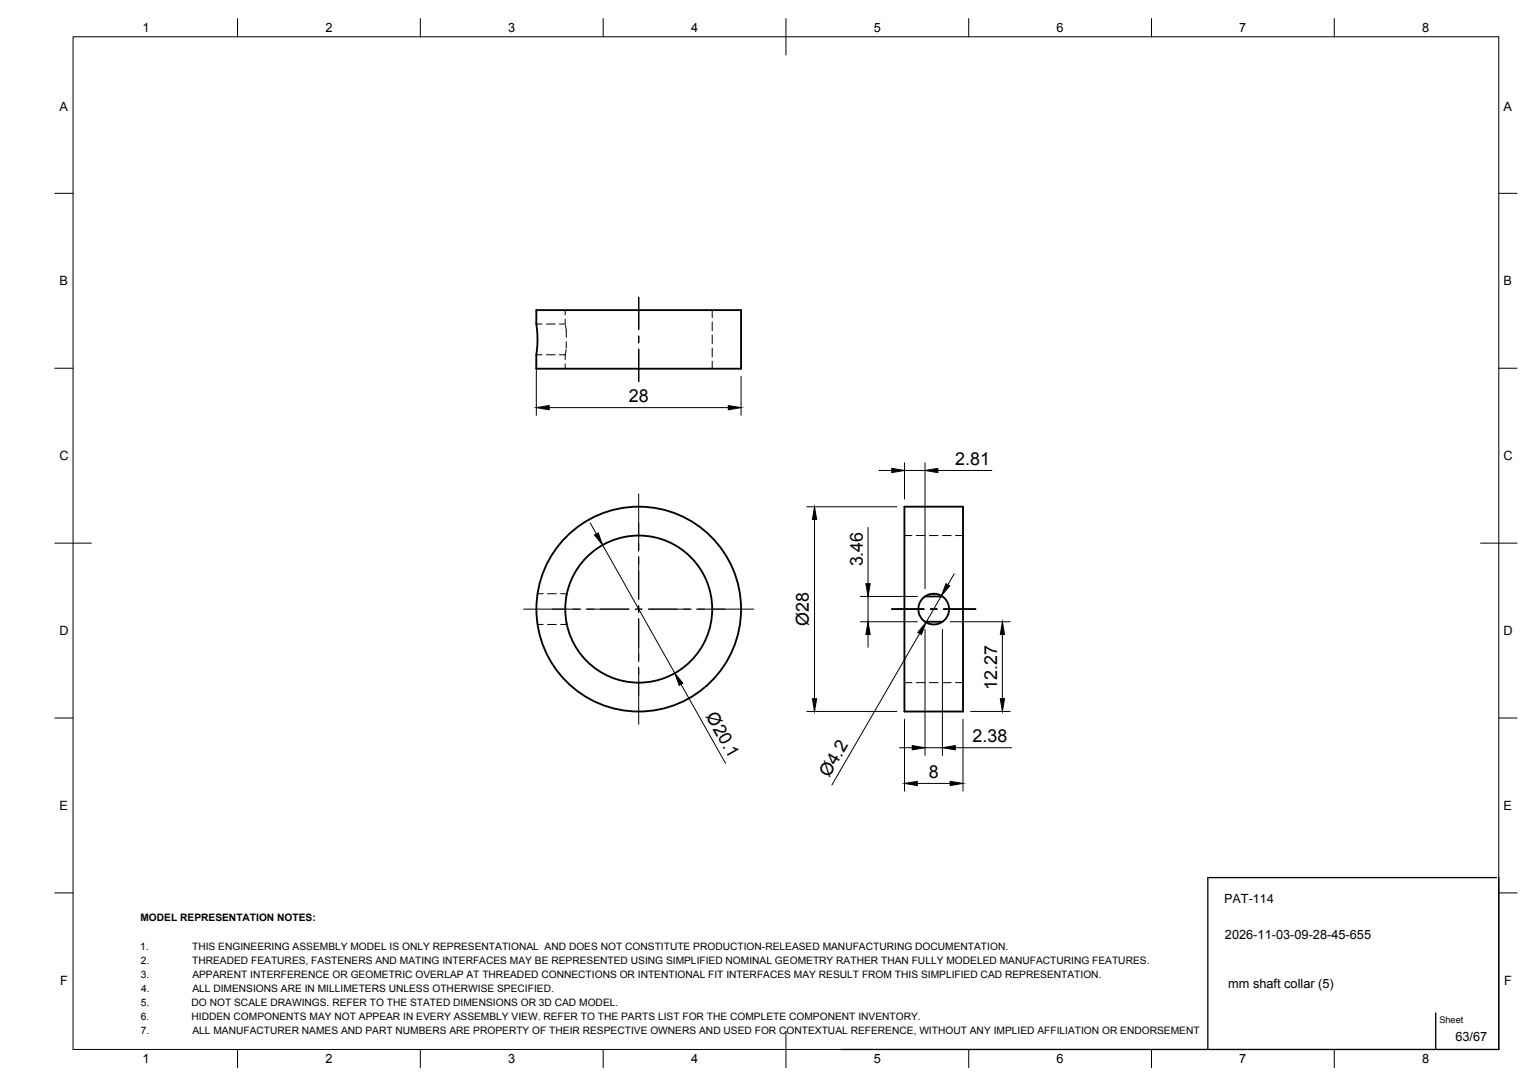
ISO-10303-21;
HEADER;
/* Generated by software containing ST-Developer
 * from STEP Tools, Inc. (www.steptools.com) 
 */

FILE_DESCRIPTION(
/* description */ ('Two-stage gear reducer in split housing'),
/* implementation_level */ '2;1');

FILE_NAME(
/* name */ 'mm shaft collar (5).step',
/* time_stamp */ '2026-10-28T03:22:31-07:00',
/* author */ (''),
/* organization */ (''),
/* preprocessor_version */ 'ST-DEVELOPER v20.2',
/* originating_system */ 'Autodesk Translation Framework v15.17.0.0',
/* authorisation */ '');

FILE_SCHEMA (('AUTOMOTIVE_DESIGN { 1 0 10303 214 3 1 1 }'));
ENDSEC;

DATA;
#10=MECHANICAL_DESIGN_GEOMETRIC_PRESENTATION_REPRESENTATION('',(#1297),#73366);
#983=B_SPLINE_CURVE_WITH_KNOTS('',3,(#49393,#49394,#49395,#49396,#49397,
#49398,#49399,#49400,#49401,#49402,#49403,#49404,#49405,#49406),
 .UNSPECIFIED.,.F.,.F.,(4,2,2,2,2,2,4),(0.756005737987027,0.79356882756465,
0.872922520054205,0.95227621254376,1.03162990503331,1.11098359752287,1.14854668710049),
 .UNSPECIFIED.);
#984=B_SPLINE_CURVE_WITH_KNOTS('',3,(#49412,#49413,#49414,#49415,#49416,
#49417,#49418,#49419,#49420,#49421,#49422,#49423,#49424,#49425,#49426,#49427,
#49428,#49429),.UNSPECIFIED.,.F.,.F.,(4,2,2,2,2,2,2,2,4),(0.,0.0792334805614376,
0.158466961122875,0.237699060165218,0.316931159207561,0.396163258249904,
0.475395357292247,0.554628837853685,0.633862318415122),.UNSPECIFIED.);
#985=B_SPLINE_CURVE_WITH_KNOTS('',3,(#49430,#49431,#49432,#49433,#49434,
#49435,#49436,#49437,#49438,#49439,#49440,#49441,#49442,#49443,#49444,#49445,
#49446,#49447),.UNSPECIFIED.,.F.,.F.,(4,2,2,2,2,2,2,2,4),(0.633862318415122,
0.71309579897656,0.792329279537998,0.871561378580341,0.950793477622684,
1.03002557666503,1.10925767570737,1.18849115626881,1.26772463683024),
 .UNSPECIFIED.);
#986=B_SPLINE_CURVE_WITH_KNOTS('',3,(#49450,#49451,#49452,#49453,#49454,
#49455,#49456,#49457,#49458,#49459,#49460,#49461,#49462,#49463),
 .UNSPECIFIED.,.F.,.F.,(4,2,2,2,2,2,4),(0.121154929624521,0.158718019202143,
0.238071711691698,0.317425404181253,0.396779096670808,0.476132789160363,
0.513695878737991),.UNSPECIFIED.);
#1170=SHAPE_REPRESENTATION_RELATIONSHIP('SRR','None',#73662,#1226);
#1226=ADVANCED_BREP_SHAPE_REPRESENTATION('',(#1366),#73358);
#1297=STYLED_ITEM('',(#73988),#1366);
#1366=MANIFOLD_SOLID_BREP('Body1',#16187);
#1586=FACE_BOUND('',#3831,.T.);
#1587=FACE_BOUND('',#3833,.T.);
#1588=FACE_BOUND('',#3835,.T.);
#1589=FACE_BOUND('',#3837,.T.);
#1925=PLANE('',#18167);
#1926=PLANE('',#18172);
#1927=PLANE('',#18179);
#1928=PLANE('',#18180);
#2702=FACE_OUTER_BOUND('',#3827,.T.);
#2703=FACE_OUTER_BOUND('',#3828,.T.);
#2704=FACE_OUTER_BOUND('',#3829,.T.);
#2705=FACE_OUTER_BOUND('',#3830,.T.);
#2706=FACE_OUTER_BOUND('',#3832,.T.);
#2707=FACE_OUTER_BOUND('',#3834,.T.);
#2708=FACE_OUTER_BOUND('',#3836,.T.);
#3827=EDGE_LOOP('',(#13739,#13740));
#3828=EDGE_LOOP('',(#13741,#13742,#13743,#13744,#13745,#13746,#13747,#13748,
#13749));
#3829=EDGE_LOOP('',(#13750,#13751,#13752));
#3830=EDGE_LOOP('',(#13753,#13754,#13755,#13756));
#3831=EDGE_LOOP('',(#13757,#13758,#13759,#13760));
#3832=EDGE_LOOP('',(#13761,#13762,#13763,#13764));
#3833=EDGE_LOOP('',(#13765,#13766));
#3834=EDGE_LOOP('',(#13767));
#3835=EDGE_LOOP('',(#13768));
#3836=EDGE_LOOP('',(#13769));
#3837=EDGE_LOOP('',(#13770));
#4851=LINE('',#49389,#5875);
#4852=LINE('',#49410,#5876);
#4853=LINE('',#49465,#5877);
#4854=LINE('',#49470,#5878);
#4855=LINE('',#49476,#5879);
#5875=VECTOR('',#21965,1.);
#5876=VECTOR('',#21972,0.210000000000001);
#5877=VECTOR('',#21977,1.);
#5878=VECTOR('',#21982,1.005);
#5879=VECTOR('',#21989,1.4);
#6713=CIRCLE('',#18168,0.210000000000001);
#6714=CIRCLE('',#18170,0.210000000000001);
#6715=CIRCLE('',#18171,0.210000000000001);
#6716=CIRCLE('',#18174,1.005);
#6717=CIRCLE('',#18175,1.005);
#6718=CIRCLE('',#18177,1.4);
#6719=CIRCLE('',#18178,1.4);
#7918=VERTEX_POINT('',#49387);
#7919=VERTEX_POINT('',#49388);
#7920=VERTEX_POINT('',#49392);
#7921=VERTEX_POINT('',#49407);
#7922=VERTEX_POINT('',#49409);
#7923=VERTEX_POINT('',#49411);
#7924=VERTEX_POINT('',#49448);
#7925=VERTEX_POINT('',#49467);
#7926=VERTEX_POINT('',#49469);
#7927=VERTEX_POINT('',#49473);
#7928=VERTEX_POINT('',#49475);
#9923=EDGE_CURVE('',#7918,#7919,#4851,.T.);
#9924=EDGE_CURVE('',#7918,#7919,#6713,.T.);
#9925=EDGE_CURVE('',#7920,#7918,#983,.T.);
#9926=EDGE_CURVE('',#7921,#7920,#6714,.T.);
#9927=EDGE_CURVE('',#7921,#7922,#4852,.T.);
#9928=EDGE_CURVE('',#7923,#7922,#984,.T.);
#9929=EDGE_CURVE('',#7922,#7923,#985,.T.);
#9930=EDGE_CURVE('',#7924,#7921,#6715,.T.);
#9931=EDGE_CURVE('',#7919,#7924,#986,.T.);
#9932=EDGE_CURVE('',#7924,#7920,#4853,.T.);
#9933=EDGE_CURVE('',#7925,#7925,#6716,.T.);
#9934=EDGE_CURVE('',#7925,#7926,#4854,.T.);
#9935=EDGE_CURVE('',#7926,#7926,#6717,.T.);
#9936=EDGE_CURVE('',#7927,#7927,#6718,.T.);
#9937=EDGE_CURVE('',#7927,#7928,#4855,.T.);
#9938=EDGE_CURVE('',#7928,#7928,#6719,.T.);
#13739=ORIENTED_EDGE('',*,*,#9923,.F.);
#13740=ORIENTED_EDGE('',*,*,#9924,.T.);
#13741=ORIENTED_EDGE('',*,*,#9925,.F.);
#13742=ORIENTED_EDGE('',*,*,#9926,.F.);
#13743=ORIENTED_EDGE('',*,*,#9927,.T.);
#13744=ORIENTED_EDGE('',*,*,#9928,.F.);
#13745=ORIENTED_EDGE('',*,*,#9929,.F.);
#13746=ORIENTED_EDGE('',*,*,#9927,.F.);
#13747=ORIENTED_EDGE('',*,*,#9930,.F.);
#13748=ORIENTED_EDGE('',*,*,#9931,.F.);
#13749=ORIENTED_EDGE('',*,*,#9924,.F.);
#13750=ORIENTED_EDGE('',*,*,#9932,.F.);
#13751=ORIENTED_EDGE('',*,*,#9930,.T.);
#13752=ORIENTED_EDGE('',*,*,#9926,.T.);
#13753=ORIENTED_EDGE('',*,*,#9933,.F.);
#13754=ORIENTED_EDGE('',*,*,#9934,.T.);
#13755=ORIENTED_EDGE('',*,*,#9935,.T.);
#13756=ORIENTED_EDGE('',*,*,#9934,.F.);
#13757=ORIENTED_EDGE('',*,*,#9931,.T.);
#13758=ORIENTED_EDGE('',*,*,#9932,.T.);
#13759=ORIENTED_EDGE('',*,*,#9925,.T.);
#13760=ORIENTED_EDGE('',*,*,#9923,.T.);
#13761=ORIENTED_EDGE('',*,*,#9936,.F.);
#13762=ORIENTED_EDGE('',*,*,#9937,.T.);
#13763=ORIENTED_EDGE('',*,*,#9938,.T.);
#13764=ORIENTED_EDGE('',*,*,#9937,.F.);
#13765=ORIENTED_EDGE('',*,*,#9928,.T.);
#13766=ORIENTED_EDGE('',*,*,#9929,.T.);
#13767=ORIENTED_EDGE('',*,*,#9936,.T.);
#13768=ORIENTED_EDGE('',*,*,#9933,.T.);
#13769=ORIENTED_EDGE('',*,*,#9938,.F.);
#13770=ORIENTED_EDGE('',*,*,#9935,.F.);
#15155=CYLINDRICAL_SURFACE('',#18169,0.210000000000001);
#15156=CYLINDRICAL_SURFACE('',#18173,1.005);
#15157=CYLINDRICAL_SURFACE('',#18176,1.4);
#15909=ADVANCED_FACE('',(#2702),#1925,.T.);
#15910=ADVANCED_FACE('',(#2703),#15155,.F.);
#15911=ADVANCED_FACE('',(#2704),#1926,.T.);
#15912=ADVANCED_FACE('',(#2705,#1586),#15156,.F.);
#15913=ADVANCED_FACE('',(#2706,#1587),#15157,.T.);
#15914=ADVANCED_FACE('',(#2707,#1588),#1927,.T.);
#15915=ADVANCED_FACE('',(#2708,#1589),#1928,.F.);
#16187=CLOSED_SHELL('',(#15909,#15910,#15911,#15912,#15913,#15914,#15915));
#18166=AXIS2_PLACEMENT_3D('',#49385,#21961,#21962);
#18167=AXIS2_PLACEMENT_3D('',#49386,#21963,#21964);
#18168=AXIS2_PLACEMENT_3D('',#49390,#21966,#21967);
#18169=AXIS2_PLACEMENT_3D('',#49391,#21968,#21969);
#18170=AXIS2_PLACEMENT_3D('',#49408,#21970,#21971);
#18171=AXIS2_PLACEMENT_3D('',#49449,#21973,#21974);
#18172=AXIS2_PLACEMENT_3D('',#49464,#21975,#21976);
#18173=AXIS2_PLACEMENT_3D('',#49466,#21978,#21979);
#18174=AXIS2_PLACEMENT_3D('',#49468,#21980,#21981);
#18175=AXIS2_PLACEMENT_3D('',#49471,#21983,#21984);
#18176=AXIS2_PLACEMENT_3D('',#49472,#21985,#21986);
#18177=AXIS2_PLACEMENT_3D('',#49474,#21987,#21988);
#18178=AXIS2_PLACEMENT_3D('',#49477,#21990,#21991);
#18179=AXIS2_PLACEMENT_3D('',#49478,#21992,#21993);
#18180=AXIS2_PLACEMENT_3D('',#49479,#21994,#21995);
#21961=DIRECTION('axis',(0.,0.,1.));
#21962=DIRECTION('refdir',(1.,0.,0.));
#21963=DIRECTION('center_axis',(0.,0.,1.));
#21964=DIRECTION('ref_axis',(1.,0.,0.));
#21965=DIRECTION('',(0.,1.,0.));
#21966=DIRECTION('center_axis',(0.,0.,1.));
#21967=DIRECTION('ref_axis',(1.,0.,0.));
#21968=DIRECTION('center_axis',(0.,0.,1.));
#21969=DIRECTION('ref_axis',(1.,0.,0.));
#21970=DIRECTION('center_axis',(0.,0.,1.));
#21971=DIRECTION('ref_axis',(1.,0.,0.));
#21972=DIRECTION('',(0.,0.,1.));
#21973=DIRECTION('center_axis',(0.,0.,1.));
#21974=DIRECTION('ref_axis',(1.,0.,0.));
#21975=DIRECTION('center_axis',(0.,0.,1.));
#21976=DIRECTION('ref_axis',(1.,0.,0.));
#21977=DIRECTION('',(0.,-1.,0.));
#21978=DIRECTION('center_axis',(0.,1.,0.));
#21979=DIRECTION('ref_axis',(1.,0.,0.));
#21980=DIRECTION('center_axis',(0.,-1.,0.));
#21981=DIRECTION('ref_axis',(1.,0.,0.));
#21982=DIRECTION('',(0.,-1.,0.));
#21983=DIRECTION('center_axis',(0.,-1.,0.));
#21984=DIRECTION('ref_axis',(1.,0.,0.));
#21985=DIRECTION('center_axis',(0.,1.,0.));
#21986=DIRECTION('ref_axis',(1.,0.,0.));
#21987=DIRECTION('center_axis',(0.,1.,0.));
#21988=DIRECTION('ref_axis',(1.,0.,0.));
#21989=DIRECTION('',(0.,-1.,0.));
#21990=DIRECTION('center_axis',(0.,1.,0.));
#21991=DIRECTION('ref_axis',(1.,0.,0.));
#21992=DIRECTION('center_axis',(0.,1.,0.));
#21993=DIRECTION('ref_axis',(1.,0.,0.));
#21994=DIRECTION('center_axis',(0.,1.,0.));
#21995=DIRECTION('ref_axis',(1.,0.,0.));
#49385=CARTESIAN_POINT('',(0.,0.,0.));
#49386=CARTESIAN_POINT('Origin',(12.,8.2,10.99));
#49387=CARTESIAN_POINT('',(12.1729884389201,8.08094119100208,10.99));
#49388=CARTESIAN_POINT('',(12.1729884389201,8.31905880899792,10.99));
#49389=CARTESIAN_POINT('',(12.1729884389201,7.8,10.99));
#49390=CARTESIAN_POINT('Origin',(12.,8.2,10.99));
#49391=CARTESIAN_POINT('Origin',(12.,8.2,10.99));
#49392=CARTESIAN_POINT('',(11.8270115610799,8.08094119100208,10.99));
#49393=CARTESIAN_POINT('Ctrl Pts',(11.8270115610799,8.08094119100208,10.99));
#49394=CARTESIAN_POINT('Ctrl Pts',(11.8344051346887,8.0701985776047,10.9912919219764));
#49395=CARTESIAN_POINT('Ctrl Pts',(11.8427028612744,8.06031229062725,10.992653949439));
#49396=CARTESIAN_POINT('Ctrl Pts',(11.8701079261549,8.03290722574673,10.9967480843909));
#49397=CARTESIAN_POINT('Ctrl Pts',(11.8936698322407,8.01675794366705,10.9996958932764));
#49398=CARTESIAN_POINT('Ctrl Pts',(11.9453870953676,7.99530220603509,11.0038502947236));
#49399=CARTESIAN_POINT('Ctrl Pts',(11.9735487691701,7.99,11.005));
#49400=CARTESIAN_POINT('Ctrl Pts',(12.0264512308299,7.99,11.005));
#49401=CARTESIAN_POINT('Ctrl Pts',(12.0546129046324,7.99530220603509,11.0038502947236));
#49402=CARTESIAN_POINT('Ctrl Pts',(12.1063301677593,8.01675794366705,10.9996958932764));
#49403=CARTESIAN_POINT('Ctrl Pts',(12.1298920738451,8.03290722574673,10.9967480843909));
#49404=CARTESIAN_POINT('Ctrl Pts',(12.1572971387256,8.06031229062725,10.992653949439));
#49405=CARTESIAN_POINT('Ctrl Pts',(12.1655948653113,8.0701985776047,10.9912919219764));
#49406=CARTESIAN_POINT('Ctrl Pts',(12.1729884389201,8.08094119100208,10.99));
#49407=CARTESIAN_POINT('',(11.79,8.2,10.99));
#49408=CARTESIAN_POINT('Origin',(12.,8.2,10.99));
#49409=CARTESIAN_POINT('',(11.79,8.2,11.38416039533));
#49410=CARTESIAN_POINT('',(11.79,8.2,10.99));
#49411=CARTESIAN_POINT('',(12.21,8.2,11.38416039533));
#49412=CARTESIAN_POINT('Ctrl Pts',(12.21,8.2,11.38416039533));
#49413=CARTESIAN_POINT('Ctrl Pts',(12.21,8.17358883981285,11.38416039533));
#49414=CARTESIAN_POINT('Ctrl Pts',(12.2047135491119,8.1454449403829,11.3849944296993));
#49415=CARTESIAN_POINT('Ctrl Pts',(12.1832699958585,8.09371735000826,11.3879947099895));
#49416=CARTESIAN_POINT('Ctrl Pts',(12.1671150376064,8.07013018950807,11.3901162943626));
#49417=CARTESIAN_POINT('Ctrl Pts',(12.1298701351968,8.03288528709843,11.394089123191));
#49418=CARTESIAN_POINT('Ctrl Pts',(12.1062828345902,8.01673007414492,11.3962002442067));
#49419=CARTESIAN_POINT('Ctrl Pts',(12.0545547656039,7.99528633552708,11.3991765222353));
#49420=CARTESIAN_POINT('Ctrl Pts',(12.0264106996808,7.99,11.4));
#49421=CARTESIAN_POINT('Ctrl Pts',(11.9735893003192,7.99,11.4));
#49422=CARTESIAN_POINT('Ctrl Pts',(11.9454452343961,7.99528633552708,11.3991765222353));
#49423=CARTESIAN_POINT('Ctrl Pts',(11.8937171654098,8.01673007414492,11.3962002442067));
#49424=CARTESIAN_POINT('Ctrl Pts',(11.8701298648032,8.03288528709843,11.394089123191));
#49425=CARTESIAN_POINT('Ctrl Pts',(11.8328849623936,8.07013018950807,11.3901162943626));
#49426=CARTESIAN_POINT('Ctrl Pts',(11.8167300041415,8.09371735000826,11.3879947099895));
#49427=CARTESIAN_POINT('Ctrl Pts',(11.7952864508881,8.1454449403829,11.3849944296993));
#49428=CARTESIAN_POINT('Ctrl Pts',(11.79,8.17358883981285,11.38416039533));
#49429=CARTESIAN_POINT('Ctrl Pts',(11.79,8.2,11.38416039533));
#49430=CARTESIAN_POINT('Ctrl Pts',(11.79,8.2,11.38416039533));
#49431=CARTESIAN_POINT('Ctrl Pts',(11.79,8.22641116018714,11.38416039533));
#49432=CARTESIAN_POINT('Ctrl Pts',(11.7952864508881,8.2545550596171,11.3849944296993));
#49433=CARTESIAN_POINT('Ctrl Pts',(11.8167300041415,8.30628264999174,11.3879947099895));
#49434=CARTESIAN_POINT('Ctrl Pts',(11.8328849623936,8.32986981049192,11.3901162943626));
#49435=CARTESIAN_POINT('Ctrl Pts',(11.8701298648032,8.36711471290156,11.394089123191));
#49436=CARTESIAN_POINT('Ctrl Pts',(11.8937171654098,8.38326992585508,11.3962002442067));
#49437=CARTESIAN_POINT('Ctrl Pts',(11.9454452343961,8.40471366447292,11.3991765222353));
#49438=CARTESIAN_POINT('Ctrl Pts',(11.9735893003192,8.41,11.4));
#49439=CARTESIAN_POINT('Ctrl Pts',(12.0264106996808,8.41,11.4));
#49440=CARTESIAN_POINT('Ctrl Pts',(12.0545547656039,8.40471366447292,11.3991765222353));
#49441=CARTESIAN_POINT('Ctrl Pts',(12.1062828345902,8.38326992585508,11.3962002442067));
#49442=CARTESIAN_POINT('Ctrl Pts',(12.1298701351968,8.36711471290156,11.394089123191));
#49443=CARTESIAN_POINT('Ctrl Pts',(12.1671150376064,8.32986981049192,11.3901162943626));
#49444=CARTESIAN_POINT('Ctrl Pts',(12.1832699958585,8.30628264999174,11.3879947099895));
#49445=CARTESIAN_POINT('Ctrl Pts',(12.2047135491119,8.2545550596171,11.3849944296993));
#49446=CARTESIAN_POINT('Ctrl Pts',(12.21,8.22641116018714,11.38416039533));
#49447=CARTESIAN_POINT('Ctrl Pts',(12.21,8.2,11.38416039533));
#49448=CARTESIAN_POINT('',(11.8270115610799,8.31905880899792,10.99));
#49449=CARTESIAN_POINT('Origin',(12.,8.2,10.99));
#49450=CARTESIAN_POINT('Ctrl Pts',(12.1729884389201,8.31905880899792,10.99));
#49451=CARTESIAN_POINT('Ctrl Pts',(12.1655948653113,8.32980142239529,10.9912919219764));
#49452=CARTESIAN_POINT('Ctrl Pts',(12.1572971387256,8.33968770937275,10.992653949439));
#49453=CARTESIAN_POINT('Ctrl Pts',(12.1298920738451,8.36709277425327,10.9967480843909));
#49454=CARTESIAN_POINT('Ctrl Pts',(12.1063301677593,8.38324205633295,10.9996958932764));
#49455=CARTESIAN_POINT('Ctrl Pts',(12.0546129046324,8.40469779396491,11.0038502947236));
#49456=CARTESIAN_POINT('Ctrl Pts',(12.0264512308299,8.41,11.005));
#49457=CARTESIAN_POINT('Ctrl Pts',(11.9735487691701,8.41,11.005));
#49458=CARTESIAN_POINT('Ctrl Pts',(11.9453870953676,8.40469779396491,11.0038502947236));
#49459=CARTESIAN_POINT('Ctrl Pts',(11.8936698322407,8.38324205633295,10.9996958932764));
#49460=CARTESIAN_POINT('Ctrl Pts',(11.8701079261549,8.36709277425327,10.9967480843909));
#49461=CARTESIAN_POINT('Ctrl Pts',(11.8427028612744,8.33968770937274,10.992653949439));
#49462=CARTESIAN_POINT('Ctrl Pts',(11.8344051346887,8.3298014223953,10.9912919219764));
#49463=CARTESIAN_POINT('Ctrl Pts',(11.8270115610799,8.31905880899792,10.99));
#49464=CARTESIAN_POINT('Origin',(12.,8.2,10.99));
#49465=CARTESIAN_POINT('',(11.8270115610799,7.8,10.99));
#49466=CARTESIAN_POINT('Origin',(12.,7.8,10.));
#49467=CARTESIAN_POINT('',(10.995,8.6,10.));
#49468=CARTESIAN_POINT('Origin',(12.,8.6,10.));
#49469=CARTESIAN_POINT('',(10.995,7.8,10.));
#49470=CARTESIAN_POINT('',(10.995,7.8,10.));
#49471=CARTESIAN_POINT('Origin',(12.,7.8,10.));
#49472=CARTESIAN_POINT('Origin',(12.,7.8,10.));
#49473=CARTESIAN_POINT('',(10.6,8.6,10.));
#49474=CARTESIAN_POINT('Origin',(12.,8.6,10.));
#49475=CARTESIAN_POINT('',(10.6,7.8,10.));
#49476=CARTESIAN_POINT('',(10.6,7.8,10.));
#49477=CARTESIAN_POINT('Origin',(12.,7.8,10.));
#49478=CARTESIAN_POINT('Origin',(12.,8.6,10.));
#49479=CARTESIAN_POINT('Origin',(12.,7.8,10.));
#73294=UNCERTAINTY_MEASURE_WITH_UNIT(LENGTH_MEASURE(0.001),#73367,
'DISTANCE_ACCURACY_VALUE',
'Maximum model space distance between geometric entities at asserted c
onnectivities');
#73302=UNCERTAINTY_MEASURE_WITH_UNIT(LENGTH_MEASURE(0.001),#73367,
'DISTANCE_ACCURACY_VALUE',
'Maximum model space distance between geometric entities at asserted c
onnectivities');
#73358=(
GEOMETRIC_REPRESENTATION_CONTEXT(3)
GLOBAL_UNCERTAINTY_ASSIGNED_CONTEXT((#73294))
GLOBAL_UNIT_ASSIGNED_CONTEXT((#73367,#73369,#73370))
REPRESENTATION_CONTEXT('','3D')
);
#73366=(
GEOMETRIC_REPRESENTATION_CONTEXT(3)
GLOBAL_UNCERTAINTY_ASSIGNED_CONTEXT((#73302))
GLOBAL_UNIT_ASSIGNED_CONTEXT((#73367,#73369,#73370))
REPRESENTATION_CONTEXT('','3D')
);
#73367=(
LENGTH_UNIT()
NAMED_UNIT(*)
SI_UNIT(.CENTI.,.METRE.)
);
#73369=(
NAMED_UNIT(*)
PLANE_ANGLE_UNIT()
SI_UNIT($,.RADIAN.)
);
#73370=(
NAMED_UNIT(*)
SI_UNIT($,.STERADIAN.)
SOLID_ANGLE_UNIT()
);
#73426=SHAPE_DEFINITION_REPRESENTATION(#73559,#73662);
#73559=PRODUCT_DEFINITION_SHAPE('',$,#73726);
#73662=SHAPE_REPRESENTATION('',(#18166),#73358);
#73670=PRODUCT_DEFINITION_CONTEXT('part definition',#73861,'design');
#73726=PRODUCT_DEFINITION('mm shaft collar (5)','mm shaft collar (5)',#73789,
#73670);
#73789=PRODUCT_DEFINITION_FORMATION('',$,#73918);
#73861=APPLICATION_CONTEXT(
'Core Data for Automotive Mechanical Design Process');
#73862=PRODUCT_CONTEXT('part definition',#73861,'mechanical');
#73918=PRODUCT('mm shaft collar (5)','mm shaft collar (5)',
'mm shaft collar (5)',(#73862));
#73982=COLOUR_RGB('Grey',0.48,0.52,0.57);
#73983=FILL_AREA_STYLE_COLOUR('',#73982);
#73984=FILL_AREA_STYLE('',(#73983));
#73985=SURFACE_STYLE_FILL_AREA(#73984);
#73986=SURFACE_SIDE_STYLE('',(#73985));
#73987=SURFACE_STYLE_USAGE(.BOTH.,#73986);
#73988=PRESENTATION_STYLE_ASSIGNMENT((#73987));
ENDSEC;
END-ISO-10303-21;
